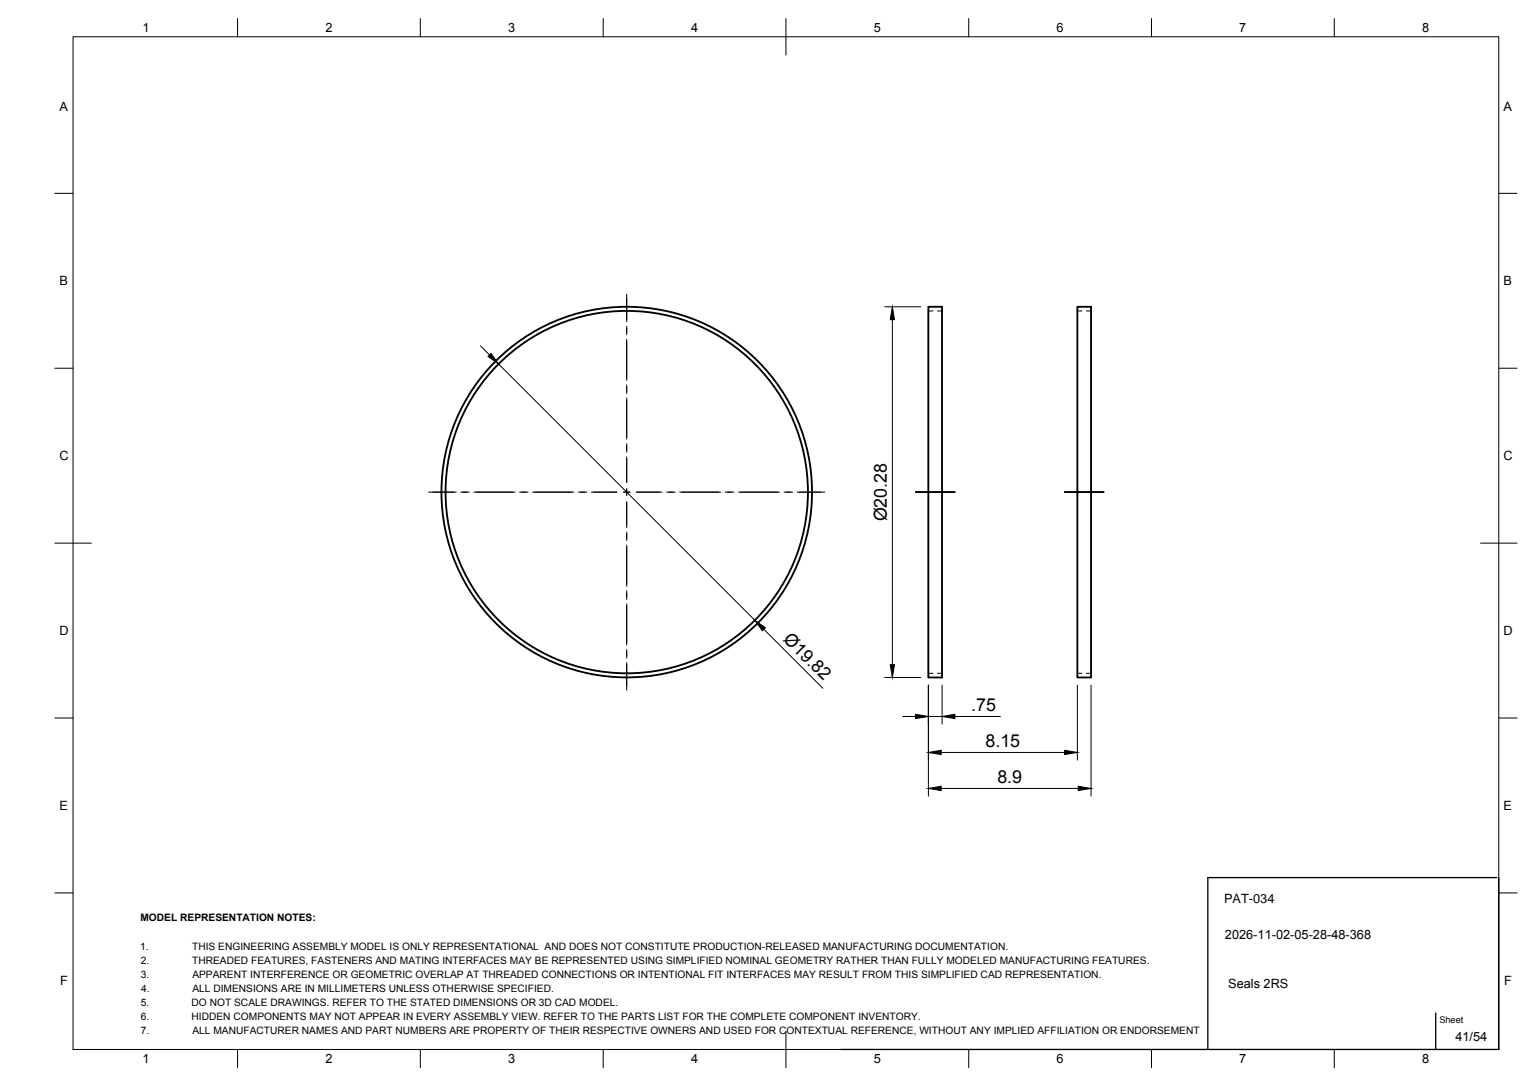
ISO-10303-21;
HEADER;
/* Generated by software containing ST-Developer
 * from STEP Tools, Inc. (www.steptools.com) 
 */

FILE_DESCRIPTION(
/* description */ ('Fatigue rig crank-slider'),
/* implementation_level */ '2;1');

FILE_NAME(
/* name */ 'Seals 2RS.step',
/* time_stamp */ '2026-10-28T03:24:50-07:00',
/* author */ (''),
/* organization */ (''),
/* preprocessor_version */ 'ST-DEVELOPER v20.2',
/* originating_system */ 'Autodesk Translation Framework v15.17.0.0',
/* authorisation */ '');

FILE_SCHEMA (('AUTOMOTIVE_DESIGN { 1 0 10303 214 3 1 1 }'));
ENDSEC;

DATA;
#10=MECHANICAL_DESIGN_GEOMETRIC_PRESENTATION_REPRESENTATION('',(#631,#632),#16911);
#523=SHAPE_REPRESENTATION_RELATIONSHIP('SRR','None',#17166,#573);
#573=ADVANCED_BREP_SHAPE_REPRESENTATION('',(#688,#689),#16895);
#631=STYLED_ITEM('',(#17487),#688);
#632=STYLED_ITEM('',(#17487),#689);
#688=MANIFOLD_SOLID_BREP('Body1',#8924);
#689=MANIFOLD_SOLID_BREP('Body2',#8925);
#859=FACE_BOUND('',#2268,.T.);
#860=FACE_BOUND('',#2271,.T.);
#861=FACE_BOUND('',#2274,.T.);
#862=FACE_BOUND('',#2277,.T.);
#1107=PLANE('',#10219);
#1108=PLANE('',#10224);
#1109=PLANE('',#10227);
#1110=PLANE('',#10232);
#1585=FACE_OUTER_BOUND('',#2267,.T.);
#1586=FACE_OUTER_BOUND('',#2269,.T.);
#1587=FACE_OUTER_BOUND('',#2270,.T.);
#1588=FACE_OUTER_BOUND('',#2272,.T.);
#1589=FACE_OUTER_BOUND('',#2273,.T.);
#1590=FACE_OUTER_BOUND('',#2275,.T.);
#1591=FACE_OUTER_BOUND('',#2276,.T.);
#1592=FACE_OUTER_BOUND('',#2278,.T.);
#2267=EDGE_LOOP('',(#7528));
#2268=EDGE_LOOP('',(#7529));
#2269=EDGE_LOOP('',(#7530,#7531,#7532,#7533));
#2270=EDGE_LOOP('',(#7534));
#2271=EDGE_LOOP('',(#7535));
#2272=EDGE_LOOP('',(#7536,#7537,#7538,#7539));
#2273=EDGE_LOOP('',(#7540));
#2274=EDGE_LOOP('',(#7541));
#2275=EDGE_LOOP('',(#7542,#7543,#7544,#7545));
#2276=EDGE_LOOP('',(#7546));
#2277=EDGE_LOOP('',(#7547));
#2278=EDGE_LOOP('',(#7548,#7549,#7550,#7551));
#2859=LINE('',#15989,#3505);
#2860=LINE('',#15994,#3506);
#2861=LINE('',#16003,#3507);
#2862=LINE('',#16008,#3508);
#3505=VECTOR('',#12427,1.013815);
#3506=VECTOR('',#12434,0.991185);
#3507=VECTOR('',#12445,1.013815);
#3508=VECTOR('',#12452,0.991185);
#4065=CIRCLE('',#10220,1.013815);
#4066=CIRCLE('',#10221,0.991185);
#4067=CIRCLE('',#10223,1.013815);
#4068=CIRCLE('',#10225,0.991185);
#4069=CIRCLE('',#10228,1.013815);
#4070=CIRCLE('',#10229,0.991185);
#4071=CIRCLE('',#10231,1.013815);
#4072=CIRCLE('',#10233,0.991185);
#4677=VERTEX_POINT('',#15982);
#4678=VERTEX_POINT('',#15984);
#4679=VERTEX_POINT('',#15987);
#4680=VERTEX_POINT('',#15991);
#4681=VERTEX_POINT('',#15996);
#4682=VERTEX_POINT('',#15998);
#4683=VERTEX_POINT('',#16001);
#4684=VERTEX_POINT('',#16005);
#5662=EDGE_CURVE('',#4677,#4677,#4065,.T.);
#5663=EDGE_CURVE('',#4678,#4678,#4066,.T.);
#5664=EDGE_CURVE('',#4679,#4679,#4067,.T.);
#5665=EDGE_CURVE('',#4679,#4677,#2859,.T.);
#5666=EDGE_CURVE('',#4680,#4680,#4068,.T.);
#5667=EDGE_CURVE('',#4680,#4678,#2860,.T.);
#5668=EDGE_CURVE('',#4681,#4681,#4069,.T.);
#5669=EDGE_CURVE('',#4682,#4682,#4070,.T.);
#5670=EDGE_CURVE('',#4683,#4683,#4071,.T.);
#5671=EDGE_CURVE('',#4683,#4681,#2861,.T.);
#5672=EDGE_CURVE('',#4684,#4684,#4072,.T.);
#5673=EDGE_CURVE('',#4684,#4682,#2862,.T.);
#7528=ORIENTED_EDGE('',*,*,#5662,.F.);
#7529=ORIENTED_EDGE('',*,*,#5663,.T.);
#7530=ORIENTED_EDGE('',*,*,#5664,.F.);
#7531=ORIENTED_EDGE('',*,*,#5665,.T.);
#7532=ORIENTED_EDGE('',*,*,#5662,.T.);
#7533=ORIENTED_EDGE('',*,*,#5665,.F.);
#7534=ORIENTED_EDGE('',*,*,#5664,.T.);
#7535=ORIENTED_EDGE('',*,*,#5666,.F.);
#7536=ORIENTED_EDGE('',*,*,#5666,.T.);
#7537=ORIENTED_EDGE('',*,*,#5667,.T.);
#7538=ORIENTED_EDGE('',*,*,#5663,.F.);
#7539=ORIENTED_EDGE('',*,*,#5667,.F.);
#7540=ORIENTED_EDGE('',*,*,#5668,.F.);
#7541=ORIENTED_EDGE('',*,*,#5669,.T.);
#7542=ORIENTED_EDGE('',*,*,#5670,.F.);
#7543=ORIENTED_EDGE('',*,*,#5671,.T.);
#7544=ORIENTED_EDGE('',*,*,#5668,.T.);
#7545=ORIENTED_EDGE('',*,*,#5671,.F.);
#7546=ORIENTED_EDGE('',*,*,#5670,.T.);
#7547=ORIENTED_EDGE('',*,*,#5672,.F.);
#7548=ORIENTED_EDGE('',*,*,#5672,.T.);
#7549=ORIENTED_EDGE('',*,*,#5673,.T.);
#7550=ORIENTED_EDGE('',*,*,#5669,.F.);
#7551=ORIENTED_EDGE('',*,*,#5673,.F.);
#8321=CYLINDRICAL_SURFACE('',#10222,1.013815);
#8322=CYLINDRICAL_SURFACE('',#10226,0.991185);
#8323=CYLINDRICAL_SURFACE('',#10230,1.013815);
#8324=CYLINDRICAL_SURFACE('',#10234,0.991185);
#8723=ADVANCED_FACE('',(#1585,#859),#1107,.T.);
#8724=ADVANCED_FACE('',(#1586),#8321,.T.);
#8725=ADVANCED_FACE('',(#1587,#860),#1108,.T.);
#8726=ADVANCED_FACE('',(#1588),#8322,.F.);
#8727=ADVANCED_FACE('',(#1589,#861),#1109,.T.);
#8728=ADVANCED_FACE('',(#1590),#8323,.T.);
#8729=ADVANCED_FACE('',(#1591,#862),#1110,.T.);
#8730=ADVANCED_FACE('',(#1592),#8324,.F.);
#8924=CLOSED_SHELL('',(#8723,#8724,#8725,#8726));
#8925=CLOSED_SHELL('',(#8727,#8728,#8729,#8730));
#10218=AXIS2_PLACEMENT_3D('',#15980,#12415,#12416);
#10219=AXIS2_PLACEMENT_3D('',#15981,#12417,#12418);
#10220=AXIS2_PLACEMENT_3D('',#15983,#12419,#12420);
#10221=AXIS2_PLACEMENT_3D('',#15985,#12421,#12422);
#10222=AXIS2_PLACEMENT_3D('',#15986,#12423,#12424);
#10223=AXIS2_PLACEMENT_3D('',#15988,#12425,#12426);
#10224=AXIS2_PLACEMENT_3D('',#15990,#12428,#12429);
#10225=AXIS2_PLACEMENT_3D('',#15992,#12430,#12431);
#10226=AXIS2_PLACEMENT_3D('',#15993,#12432,#12433);
#10227=AXIS2_PLACEMENT_3D('',#15995,#12435,#12436);
#10228=AXIS2_PLACEMENT_3D('',#15997,#12437,#12438);
#10229=AXIS2_PLACEMENT_3D('',#15999,#12439,#12440);
#10230=AXIS2_PLACEMENT_3D('',#16000,#12441,#12442);
#10231=AXIS2_PLACEMENT_3D('',#16002,#12443,#12444);
#10232=AXIS2_PLACEMENT_3D('',#16004,#12446,#12447);
#10233=AXIS2_PLACEMENT_3D('',#16006,#12448,#12449);
#10234=AXIS2_PLACEMENT_3D('',#16007,#12450,#12451);
#12415=DIRECTION('axis',(0.,0.,1.));
#12416=DIRECTION('refdir',(1.,0.,0.));
#12417=DIRECTION('center_axis',(0.,1.,0.));
#12418=DIRECTION('ref_axis',(0.,0.,1.));
#12419=DIRECTION('center_axis',(0.,-1.,0.));
#12420=DIRECTION('ref_axis',(1.,0.,0.));
#12421=DIRECTION('center_axis',(0.,-1.,0.));
#12422=DIRECTION('ref_axis',(1.,0.,0.));
#12423=DIRECTION('center_axis',(0.,-1.,0.));
#12424=DIRECTION('ref_axis',(1.,0.,0.));
#12425=DIRECTION('center_axis',(0.,-1.,0.));
#12426=DIRECTION('ref_axis',(1.,0.,0.));
#12427=DIRECTION('',(0.,1.,0.));
#12428=DIRECTION('center_axis',(0.,-1.,0.));
#12429=DIRECTION('ref_axis',(0.,0.,-1.));
#12430=DIRECTION('center_axis',(0.,-1.,0.));
#12431=DIRECTION('ref_axis',(1.,0.,0.));
#12432=DIRECTION('center_axis',(0.,-1.,0.));
#12433=DIRECTION('ref_axis',(1.,0.,0.));
#12434=DIRECTION('',(0.,1.,0.));
#12435=DIRECTION('center_axis',(0.,1.,0.));
#12436=DIRECTION('ref_axis',(0.,0.,1.));
#12437=DIRECTION('center_axis',(0.,-1.,0.));
#12438=DIRECTION('ref_axis',(1.,0.,0.));
#12439=DIRECTION('center_axis',(0.,-1.,0.));
#12440=DIRECTION('ref_axis',(1.,0.,0.));
#12441=DIRECTION('center_axis',(0.,-1.,0.));
#12442=DIRECTION('ref_axis',(1.,0.,0.));
#12443=DIRECTION('center_axis',(0.,-1.,0.));
#12444=DIRECTION('ref_axis',(1.,0.,0.));
#12445=DIRECTION('',(0.,1.,0.));
#12446=DIRECTION('center_axis',(0.,-1.,0.));
#12447=DIRECTION('ref_axis',(0.,0.,-1.));
#12448=DIRECTION('center_axis',(0.,-1.,0.));
#12449=DIRECTION('ref_axis',(1.,0.,0.));
#12450=DIRECTION('center_axis',(0.,-1.,0.));
#12451=DIRECTION('ref_axis',(1.,0.,0.));
#12452=DIRECTION('',(0.,1.,0.));
#15980=CARTESIAN_POINT('',(0.,0.,0.));
#15981=CARTESIAN_POINT('Origin',(1.013815,0.445,0.));
#15982=CARTESIAN_POINT('',(-1.013815,0.445,-1.24156529467757E-16));
#15983=CARTESIAN_POINT('Origin',(0.,0.445,0.));
#15984=CARTESIAN_POINT('',(-0.991185,0.445,-1.21385153761287E-16));
#15985=CARTESIAN_POINT('Origin',(0.,0.445,0.));
#15986=CARTESIAN_POINT('Origin',(0.,0.4075,0.));
#15987=CARTESIAN_POINT('',(-1.013815,0.37,-1.24156529467757E-16));
#15988=CARTESIAN_POINT('Origin',(0.,0.37,0.));
#15989=CARTESIAN_POINT('',(-1.013815,0.4075,-1.24156529467757E-16));
#15990=CARTESIAN_POINT('Origin',(0.991185,0.37,0.));
#15991=CARTESIAN_POINT('',(-0.991185,0.37,-1.21385153761287E-16));
#15992=CARTESIAN_POINT('Origin',(0.,0.37,0.));
#15993=CARTESIAN_POINT('Origin',(0.,0.4075,0.));
#15994=CARTESIAN_POINT('',(-0.991185,0.4075,-1.21385153761287E-16));
#15995=CARTESIAN_POINT('Origin',(1.013815,-0.37,0.));
#15996=CARTESIAN_POINT('',(-1.013815,-0.37,-1.24156529467757E-16));
#15997=CARTESIAN_POINT('Origin',(0.,-0.37,0.));
#15998=CARTESIAN_POINT('',(-0.991185,-0.37,-1.21385153761287E-16));
#15999=CARTESIAN_POINT('Origin',(0.,-0.37,0.));
#16000=CARTESIAN_POINT('Origin',(0.,-0.4075,0.));
#16001=CARTESIAN_POINT('',(-1.013815,-0.445,-1.24156529467757E-16));
#16002=CARTESIAN_POINT('Origin',(0.,-0.445,0.));
#16003=CARTESIAN_POINT('',(-1.013815,-0.4075,-1.24156529467757E-16));
#16004=CARTESIAN_POINT('Origin',(0.991185,-0.445,0.));
#16005=CARTESIAN_POINT('',(-0.991185,-0.445,-1.21385153761287E-16));
#16006=CARTESIAN_POINT('Origin',(0.,-0.445,0.));
#16007=CARTESIAN_POINT('Origin',(0.,-0.4075,0.));
#16008=CARTESIAN_POINT('',(-0.991185,-0.4075,-1.21385153761287E-16));
#16836=UNCERTAINTY_MEASURE_WITH_UNIT(LENGTH_MEASURE(0.001),#16912,
'DISTANCE_ACCURACY_VALUE',
'Maximum model space distance between geometric entities at asserted c
onnectivities');
#16852=UNCERTAINTY_MEASURE_WITH_UNIT(LENGTH_MEASURE(0.001),#16912,
'DISTANCE_ACCURACY_VALUE',
'Maximum model space distance between geometric entities at asserted c
onnectivities');
#16895=(
GEOMETRIC_REPRESENTATION_CONTEXT(3)
GLOBAL_UNCERTAINTY_ASSIGNED_CONTEXT((#16836))
GLOBAL_UNIT_ASSIGNED_CONTEXT((#16912,#16914,#16915))
REPRESENTATION_CONTEXT('','3D')
);
#16911=(
GEOMETRIC_REPRESENTATION_CONTEXT(3)
GLOBAL_UNCERTAINTY_ASSIGNED_CONTEXT((#16852))
GLOBAL_UNIT_ASSIGNED_CONTEXT((#16912,#16914,#16915))
REPRESENTATION_CONTEXT('','3D')
);
#16912=(
LENGTH_UNIT()
NAMED_UNIT(*)
SI_UNIT(.CENTI.,.METRE.)
);
#16914=(
NAMED_UNIT(*)
PLANE_ANGLE_UNIT()
SI_UNIT($,.RADIAN.)
);
#16915=(
NAMED_UNIT(*)
SI_UNIT($,.STERADIAN.)
SOLID_ANGLE_UNIT()
);
#16958=SHAPE_DEFINITION_REPRESENTATION(#17018,#17166);
#17018=PRODUCT_DEFINITION_SHAPE('',$,#17225);
#17166=SHAPE_REPRESENTATION('',(#10218),#16895);
#17182=PRODUCT_DEFINITION_CONTEXT('part definition',#17358,'design');
#17225=PRODUCT_DEFINITION('Seals 2RS','Seals 2RS',#17283,#17182);
#17283=PRODUCT_DEFINITION_FORMATION('',$,#17402);
#17358=APPLICATION_CONTEXT(
'Core Data for Automotive Mechanical Design Process');
#17359=PRODUCT_CONTEXT('part definition',#17358,'mechanical');
#17402=PRODUCT('Seals 2RS','Seals 2RS','Seals 2RS',(#17359));
#17481=COLOUR_RGB('Grey',0.48,0.52,0.57);
#17482=FILL_AREA_STYLE_COLOUR('',#17481);
#17483=FILL_AREA_STYLE('',(#17482));
#17484=SURFACE_STYLE_FILL_AREA(#17483);
#17485=SURFACE_SIDE_STYLE('',(#17484));
#17486=SURFACE_STYLE_USAGE(.BOTH.,#17485);
#17487=PRESENTATION_STYLE_ASSIGNMENT((#17486));
ENDSEC;
END-ISO-10303-21;
